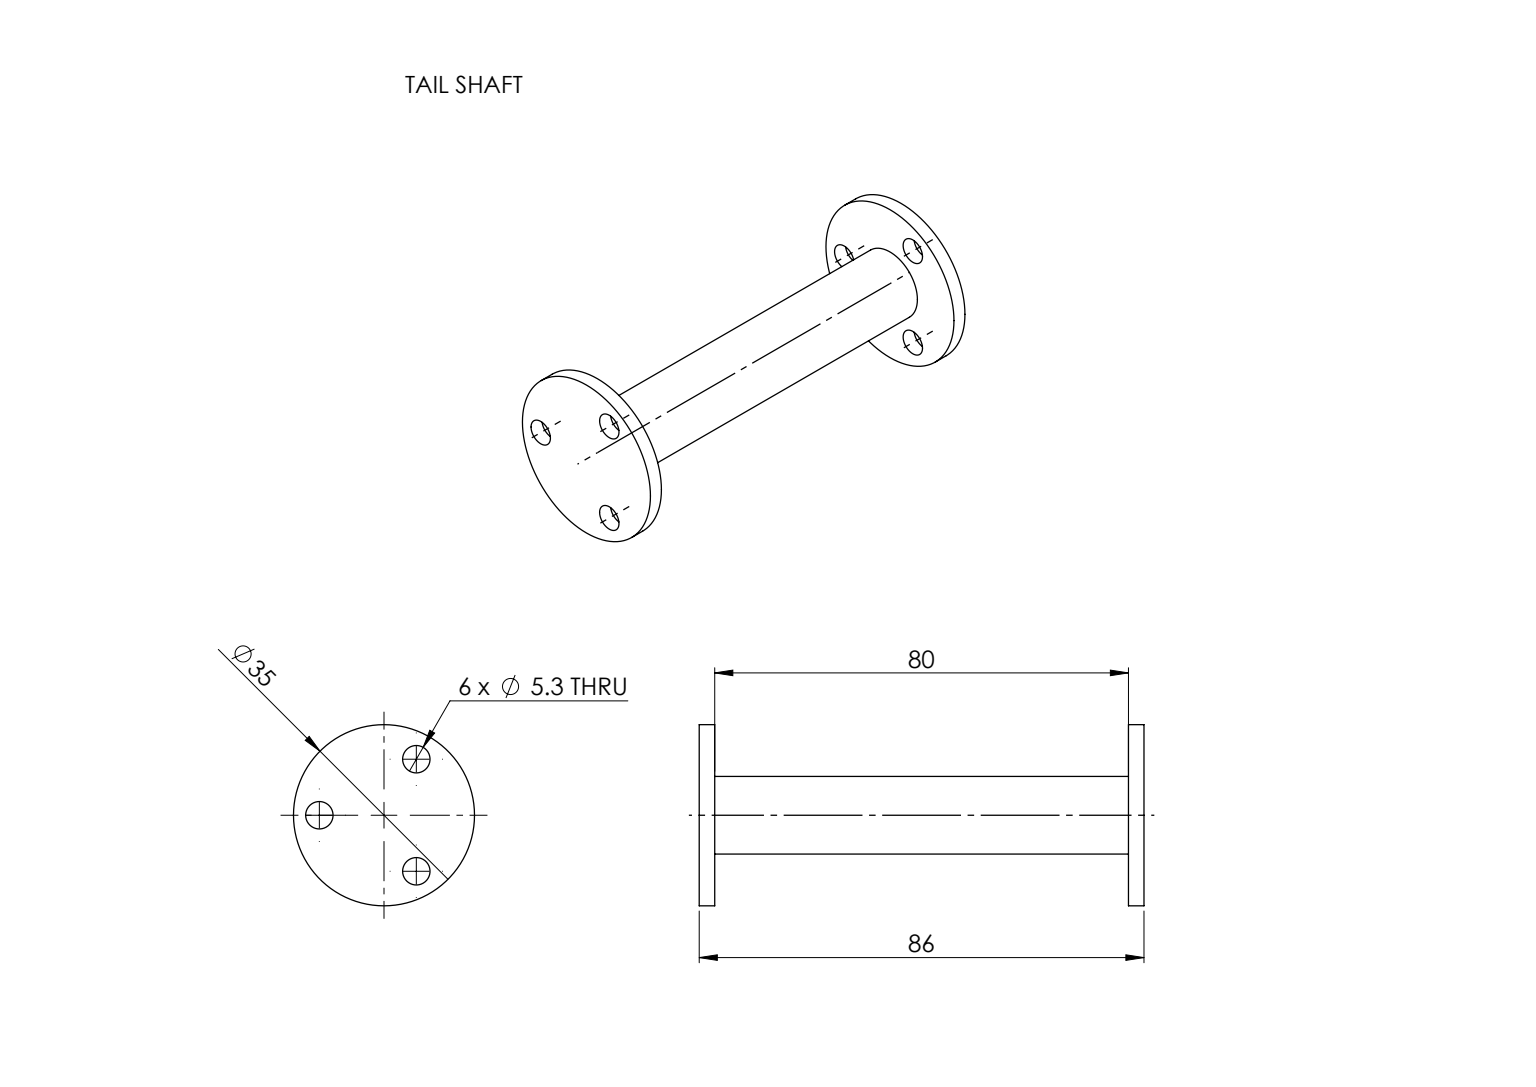
ISO-10303-21;
HEADER;
FILE_DESCRIPTION (('STEP AP214'),
    '1' );
FILE_NAME ('tail shaft.step',
    '2026-10-03T12:29:21',
    ( '' ),
    ( '' ),
    'SwSTEP 2.0',
    'SolidWorks 2026',
    '' );
FILE_SCHEMA (( 'AUTOMOTIVE_DESIGN' ));
ENDSEC;

DATA;
#68=( GEOMETRIC_REPRESENTATION_CONTEXT ( 3 ) GLOBAL_UNCERTAINTY_ASSIGNED_CONTEXT ( ( #15146 ) ) GLOBAL_UNIT_ASSIGNED_CONTEXT ( ( #18068, #7816, #19263 ) ) REPRESENTATION_CONTEXT ( 'NONE', 'WORKASPACE' ) );
#77=CARTESIAN_POINT ( 'NONE',  ( -7.500000000000000000, 0.000000000000000000, 126.0000000000000000 ) ) ;
#92=ORIENTED_EDGE ( 'NONE', *, *, #14677, .F. ) ;
#111=PLANE ( 'NONE',  #12445 ) ;
#139=ORIENTED_EDGE ( 'NONE', *, *, #678, .F. ) ;
#155=DIRECTION ( 'NONE',  ( -1.000000000000000000, 0.000000000000000000, 0.000000000000000000 ) ) ;
#169=LINE ( 'NONE', #3246, #19204 ) ;
#185=DIRECTION ( 'NONE',  ( 1.000000000000000000, 0.000000000000000000, 0.000000000000000000 ) ) ;
#190=CIRCLE ( 'NONE', #11381, 7.500000000000000000 ) ;
#191=ORIENTED_EDGE ( 'NONE', *, *, #7409, .T. ) ;
#219=CYLINDRICAL_SURFACE ( 'NONE', #12266, 2.649999999999992806 ) ;
#233=DIRECTION ( 'NONE',  ( 1.000000000000000000, 0.000000000000000000, 0.000000000000000000 ) ) ;
#258=CIRCLE ( 'NONE', #12801, 17.50000000000000355 ) ;
#306=VERTEX_POINT ( 'NONE', #7710 ) ;
#427=DIRECTION ( 'NONE',  ( -0.000000000000000000, -0.000000000000000000, 1.000000000000000000 ) ) ;
#452=DIRECTION ( 'NONE',  ( 1.000000000000000000, 0.000000000000000000, 0.000000000000000000 ) ) ;
#466=CARTESIAN_POINT ( 'NONE',  ( 6.250000000000054179, 10.82531754730546147, 126.0000000000000000 ) ) ;
#469=ORIENTED_EDGE ( 'NONE', *, *, #6864, .F. ) ;
#500=PRODUCT_CONTEXT ( 'NONE', #4657, 'mechanical' ) ;
#505=CARTESIAN_POINT ( 'NONE',  ( 6.249999999999902300, -10.82531754730554496, 126.0000000000000000 ) ) ;
#521=DIRECTION ( 'NONE',  ( -0.000000000000000000, -0.000000000000000000, 1.000000000000000000 ) ) ;
#536=CARTESIAN_POINT ( 'NONE',  ( 0.000000000000000000, 0.000000000000000000, 126.0000000000000000 ) ) ;
#624=EDGE_CURVE ( 'NONE', #15909, #5939, #1544, .T. ) ;
#627=DIRECTION ( 'NONE',  ( -0.000000000000000000, -0.000000000000000000, -1.000000000000000000 ) ) ;
#674=CARTESIAN_POINT ( 'NONE',  ( -15.14999999999999325, 0.000000000000000000, 126.0000000000000000 ) ) ;
#678=EDGE_CURVE ( 'NONE', #18976, #13722, #3439, .T. ) ;
#703=DIRECTION ( 'NONE',  ( 1.000000000000000000, 0.000000000000000000, 0.000000000000000000 ) ) ;
#725=PRODUCT_DEFINITION_CONTEXT ( 'detailed design', #8064, 'design' ) ;
#804=ORIENTED_EDGE ( 'NONE', *, *, #7119, .F. ) ;
#890=CARTESIAN_POINT ( 'NONE',  ( 0.000000000000000000, 0.000000000000000000, 46.00000000000000711 ) ) ;
#892=CIRCLE ( 'NONE', #10354, 2.649999999999987477 ) ;
#937=PLANE ( 'NONE',  #1249 ) ;
#947=ORIENTED_EDGE ( 'NONE', *, *, #16251, .T. ) ;
#971=DIRECTION ( 'NONE',  ( 1.000000000000000000, 0.000000000000000000, 0.000000000000000000 ) ) ;
#975=CARTESIAN_POINT ( 'NONE',  ( -17.50000000000000355, 0.000000000000000000, 43.00000000000000000 ) ) ;
#983=DIRECTION ( 'NONE',  ( 1.000000000000000000, 0.000000000000000000, 0.000000000000000000 ) ) ;
#1033=ORIENTED_EDGE ( 'NONE', *, *, #9203, .T. ) ;
#1066=ADVANCED_FACE ( 'NONE', ( #20892 ), #9764, .F. ) ;
#1081=DIRECTION ( 'NONE',  ( 1.000000000000000000, 0.000000000000000000, 0.000000000000000000 ) ) ;
#1082=AXIS2_PLACEMENT_3D ( 'NONE', #19195, #7847, #1081 ) ;
#1101=DIRECTION ( 'NONE',  ( 0.000000000000000000, 0.000000000000000000, 1.000000000000000000 ) ) ;
#1103=EDGE_CURVE ( 'NONE', #4018, #1536, #6170, .T. ) ;
#1116=VERTEX_POINT ( 'NONE', #13564 ) ;
#1131=CIRCLE ( 'NONE', #2124, 7.500000000000000000 ) ;
#1132=ORIENTED_EDGE ( 'NONE', *, *, #20108, .T. ) ;
#1134=EDGE_CURVE ( 'NONE', #14374, #16949, #2327, .T. ) ;
#1236=ORIENTED_EDGE ( 'NONE', *, *, #16218, .F. ) ;
#1249=AXIS2_PLACEMENT_3D ( 'NONE', #17251, #13857, #4209 ) ;
#1262=LINE ( 'NONE', #15866, #6665 ) ;
#1285=ADVANCED_FACE ( 'NONE', ( #16853 ), #219, .F. ) ;
#1288=DIRECTION ( 'NONE',  ( 0.000000000000000000, 0.000000000000000000, -1.000000000000000000 ) ) ;
#1427=DIRECTION ( 'NONE',  ( -0.000000000000000000, -0.000000000000000000, -1.000000000000000000 ) ) ;
#1474=CARTESIAN_POINT ( 'NONE',  ( -9.850000000000012079, 3.245314017740477087E-16, 129.0000000000000000 ) ) ;
#1514=CARTESIAN_POINT ( 'NONE',  ( 8.899999999999895550, -10.82531754730554496, 126.0000000000000000 ) ) ;
#1520=ORIENTED_EDGE ( 'NONE', *, *, #10012, .F. ) ;
#1526=LINE ( 'NONE', #20792, #14248 ) ;
#1536=VERTEX_POINT ( 'NONE', #9739 ) ;
#1544=LINE ( 'NONE', #17949, #7850 ) ;
#1579=FILL_AREA_STYLE ('',( #14294 ) ) ;
#1593=ORIENTED_EDGE ( 'NONE', *, *, #12629, .T. ) ;
#1629=EDGE_CURVE ( 'NONE', #9402, #16949, #2802, .T. ) ;
#1709=FACE_BOUND ( 'NONE', #7019, .T. ) ;
#1729=CARTESIAN_POINT ( 'NONE',  ( 6.250000000000054179, 10.82531754730546147, 129.0000000000000000 ) ) ;
#1812=DIRECTION ( 'NONE',  ( 1.000000000000000000, 0.000000000000000000, 0.000000000000000000 ) ) ;
#1852=DIRECTION ( 'NONE',  ( 1.000000000000000000, 0.000000000000000000, 0.000000000000000000 ) ) ;
#1863=ADVANCED_BREP_SHAPE_REPRESENTATION ( '', ( #17573, #12461 ), #3268 ) ;
#1912=EDGE_LOOP ( 'NONE', ( #92, #14154 ) ) ;
#1945=ORIENTED_EDGE ( 'NONE', *, *, #16251, .F. ) ;
#1957=PRESENTATION_STYLE_ASSIGNMENT (( #7928 ) ) ;
#1965=EDGE_LOOP ( 'NONE', ( #16112, #3916 ) ) ;
#1966=DIRECTION ( 'NONE',  ( -0.000000000000000000, -0.000000000000000000, 1.000000000000000000 ) ) ;
#2005=VERTEX_POINT ( 'NONE', #3119 ) ;
#2027=VERTEX_POINT ( 'NONE', #19327 ) ;
#2040=FACE_OUTER_BOUND ( 'NONE', #14555, .T. ) ;
#2061=DIRECTION ( 'NONE',  ( 1.000000000000000000, 0.000000000000000000, 0.000000000000000000 ) ) ;
#2124=AXIS2_PLACEMENT_3D ( 'NONE', #16818, #3872, #703 ) ;
#2156=CARTESIAN_POINT ( 'NONE',  ( 0.000000000000000000, 0.000000000000000000, 46.00000000000000711 ) ) ;
#2166=DIRECTION ( 'NONE',  ( 1.000000000000000000, 0.000000000000000000, 0.000000000000000000 ) ) ;
#2253=CARTESIAN_POINT ( 'NONE',  ( 0.000000000000000000, 0.000000000000000000, 126.0000000000000000 ) ) ;
#2257=EDGE_LOOP ( 'NONE', ( #11256, #17039 ) ) ;
#2259=ORIENTED_EDGE ( 'NONE', *, *, #8793, .T. ) ;
#2301=CARTESIAN_POINT ( 'NONE',  ( 6.249999999999902300, -10.82531754730554496, 43.00000000000000000 ) ) ;
#2327=LINE ( 'NONE', #16742, #14309 ) ;
#2341=PRESENTATION_STYLE_ASSIGNMENT (( #17191 ) ) ;
#2375=CYLINDRICAL_SURFACE ( 'NONE', #9838, 2.649999999999993694 ) ;
#2391=DIRECTION ( 'NONE',  ( 1.000000000000000000, 0.000000000000000000, 0.000000000000000000 ) ) ;
#2411=EDGE_LOOP ( 'NONE', ( #5675, #4612, #5419, #5529 ) ) ;
#2456=VERTEX_POINT ( 'NONE', #16330 ) ;
#2461=AXIS2_PLACEMENT_3D ( 'NONE', #20283, #17008, #3365 ) ;
#2485=CARTESIAN_POINT ( 'NONE',  ( 8.899999999999890221, -10.82531754730554496, 46.00000000000000711 ) ) ;
#2527=EDGE_LOOP ( 'NONE', ( #15680, #10668 ) ) ;
#2532=DIRECTION ( 'NONE',  ( 1.000000000000000000, 0.000000000000000000, 0.000000000000000000 ) ) ;
#2559=SURFACE_SIDE_STYLE ('',( #4246 ) ) ;
#2584=LINE ( 'NONE', #10646, #10427 ) ;
#2592=AXIS2_PLACEMENT_3D ( 'NONE', #20669, #17198, #983 ) ;
#2639=CIRCLE ( 'NONE', #8049, 2.649999999999987477 ) ;
#2727=ORIENTED_EDGE ( 'NONE', *, *, #20108, .F. ) ;
#2733=LINE ( 'NONE', #15662, #16649 ) ;
#2793=CARTESIAN_POINT ( 'NONE',  ( 17.50000000000000355, 2.143131898507868643E-15, 46.00000000000000711 ) ) ;
#2802=CIRCLE ( 'NONE', #2461, 2.649999999999987477 ) ;
#2831=FACE_BOUND ( 'NONE', #9265, .T. ) ;
#2836=AXIS2_PLACEMENT_3D ( 'NONE', #11379, #9882, #17856 ) ;
#2886=ORIENTED_EDGE ( 'NONE', *, *, #6253, .T. ) ;
#2893=ORIENTED_EDGE ( 'NONE', *, *, #5507, .F. ) ;
#2899=CARTESIAN_POINT ( 'NONE',  ( 6.250000000000054179, 10.82531754730546147, 43.00000000000000000 ) ) ;
#2922=CARTESIAN_POINT ( 'NONE',  ( 0.000000000000000000, 0.000000000000000000, 46.00000000000000711 ) ) ;
#2941=DIRECTION ( 'NONE',  ( 1.000000000000000000, 0.000000000000000000, 0.000000000000000000 ) ) ;
#2974=CARTESIAN_POINT ( 'NONE',  ( 6.249999999999902300, -10.82531754730554496, 129.0000000000000000 ) ) ;
#2997=EDGE_LOOP ( 'NONE', ( #1593, #20208 ) ) ;
#3000=CARTESIAN_POINT ( 'NONE',  ( -7.500000000000000000, 0.000000000000000000, 126.0000000000000000 ) ) ;
#3007=LINE ( 'NONE', #2793, #5192 ) ;
#3008=VERTEX_POINT ( 'NONE', #19183 ) ;
#3074=AXIS2_PLACEMENT_3D ( 'NONE', #466, #9793, #4921 ) ;
#3119=CARTESIAN_POINT ( 'NONE',  ( 3.600000000000066702, 10.82531754730546147, 46.00000000000000711 ) ) ;
#3210=CARTESIAN_POINT ( 'NONE',  ( -12.50000000000000533, 0.000000000000000000, 43.00000000000000000 ) ) ;
#3246=CARTESIAN_POINT ( 'NONE',  ( -17.50000000000000355, 2.143131898507868643E-15, 126.0000000000000000 ) ) ;
#3255=CIRCLE ( 'NONE', #17825, 17.50000000000000355 ) ;
#3261=CIRCLE ( 'NONE', #13748, 17.50000000000000355 ) ;
#3268=( GEOMETRIC_REPRESENTATION_CONTEXT ( 3 ) GLOBAL_UNCERTAINTY_ASSIGNED_CONTEXT ( ( #3689 ) ) GLOBAL_UNIT_ASSIGNED_CONTEXT ( ( #10185, #9871, #10087 ) ) REPRESENTATION_CONTEXT ( 'NONE', 'WORKASPACE' ) );
#3333=CYLINDRICAL_SURFACE ( 'NONE', #3074, 2.649999999999993694 ) ;
#3359=ORIENTED_EDGE ( 'NONE', *, *, #9567, .T. ) ;
#3361=DIRECTION ( 'NONE',  ( 0.000000000000000000, 0.000000000000000000, 1.000000000000000000 ) ) ;
#3365=DIRECTION ( 'NONE',  ( -1.000000000000000000, 0.000000000000000000, 0.000000000000000000 ) ) ;
#3374=EDGE_CURVE ( 'NONE', #19870, #7692, #14900, .T. ) ;
#3408=DIRECTION ( 'NONE',  ( -1.000000000000000000, 0.000000000000000000, 0.000000000000000000 ) ) ;
#3430=CARTESIAN_POINT ( 'NONE',  ( 6.250000000000054179, 10.82531754730546147, 129.0000000000000000 ) ) ;
#3439=CIRCLE ( 'NONE', #12930, 7.500000000000000000 ) ;
#3440=EDGE_LOOP ( 'NONE', ( #8664, #8272 ) ) ;
#3444=ORIENTED_EDGE ( 'NONE', *, *, #12629, .F. ) ;
#3467=VERTEX_POINT ( 'NONE', #19566 ) ;
#3481=EDGE_CURVE ( 'NONE', #14374, #14158, #20407, .T. ) ;
#3484=VECTOR ( 'NONE', #15619, 1000.000000000000000 ) ;
#3485=FACE_OUTER_BOUND ( 'NONE', #2527, .T. ) ;
#3500=EDGE_LOOP ( 'NONE', ( #2727, #10830, #6356, #14645 ) ) ;
#3548=ORIENTED_EDGE ( 'NONE', *, *, #15150, .T. ) ;
#3549=CARTESIAN_POINT ( 'NONE',  ( 0.000000000000000000, 0.000000000000000000, 43.00000000000000000 ) ) ;
#3621=DIRECTION ( 'NONE',  ( -1.000000000000000000, 0.000000000000000000, 0.000000000000000000 ) ) ;
#3658=ORIENTED_EDGE ( 'NONE', *, *, #1134, .F. ) ;
#3689=UNCERTAINTY_MEASURE_WITH_UNIT (LENGTH_MEASURE( 1.000000000000000082E-05 ), #10185, 'distance_accuracy_value', 'NONE');
#3849=EDGE_LOOP ( 'NONE', ( #17467, #17599, #2886, #15674 ) ) ;
#3872=DIRECTION ( 'NONE',  ( 0.000000000000000000, 0.000000000000000000, 1.000000000000000000 ) ) ;
#3916=ORIENTED_EDGE ( 'NONE', *, *, #3481, .T. ) ;
#3919=ADVANCED_FACE ( 'NONE', ( #17957 ), #3333, .F. ) ;
#3940=AXIS2_PLACEMENT_3D ( 'NONE', #15189, #10205, #12117 ) ;
#3947=DIRECTION ( 'NONE',  ( -1.000000000000000000, 0.000000000000000000, 0.000000000000000000 ) ) ;
#3950=FACE_OUTER_BOUND ( 'NONE', #17672, .T. ) ;
#3992=LINE ( 'NONE', #15233, #8841 ) ;
#4018=VERTEX_POINT ( 'NONE', #5639 ) ;
#4174=CARTESIAN_POINT ( 'NONE',  ( 0.000000000000000000, 0.000000000000000000, 126.0000000000000000 ) ) ;
#4194=EDGE_CURVE ( 'NONE', #3467, #17864, #1526, .T. ) ;
#4209=DIRECTION ( 'NONE',  ( 1.000000000000000000, 0.000000000000000000, -0.000000000000000000 ) ) ;
#4228=CYLINDRICAL_SURFACE ( 'NONE', #20218, 7.500000000000000000 ) ;
#4246=SURFACE_STYLE_FILL_AREA ( #20248 ) ;
#4331=AXIS2_PLACEMENT_3D ( 'NONE', #13440, #5151, #5053 ) ;
#4340=DIRECTION ( 'NONE',  ( -0.000000000000000000, -0.000000000000000000, -1.000000000000000000 ) ) ;
#4386=CYLINDRICAL_SURFACE ( 'NONE', #12999, 2.649999999999994582 ) ;
#4453=EDGE_CURVE ( 'NONE', #4018, #1116, #8381, .T. ) ;
#4486=DIRECTION ( 'NONE',  ( 0.000000000000000000, 0.000000000000000000, 1.000000000000000000 ) ) ;
#4524=ORIENTED_EDGE ( 'NONE', *, *, #7812, .T. ) ;
#4571=CIRCLE ( 'NONE', #11339, 17.50000000000000355 ) ;
#4598=CARTESIAN_POINT ( 'NONE',  ( 8.900000000000041211, 10.82531754730546147, 46.00000000000000711 ) ) ;
#4612=ORIENTED_EDGE ( 'NONE', *, *, #9538, .T. ) ;
#4657=APPLICATION_CONTEXT ( 'automotive_design' ) ;
#4703=DIRECTION ( 'NONE',  ( -1.000000000000000000, 0.000000000000000000, 0.000000000000000000 ) ) ;
#4708=CARTESIAN_POINT ( 'NONE',  ( 3.599999999999909051, -10.82531754730554496, 46.00000000000000711 ) ) ;
#4720=EDGE_CURVE ( 'NONE', #19863, #18058, #20338, .T. ) ;
#4734=EDGE_CURVE ( 'NONE', #8346, #8326, #11537, .T. ) ;
#4768=CARTESIAN_POINT ( 'NONE',  ( 3.600000000000060485, 10.82531754730546147, 46.00000000000000711 ) ) ;
#4777=ORIENTED_EDGE ( 'NONE', *, *, #13561, .T. ) ;
#4782=AXIS2_PLACEMENT_3D ( 'NONE', #2974, #5936, #17283 ) ;
#4829=VECTOR ( 'NONE', #5253, 1000.000000000000000 ) ;
#4921=DIRECTION ( 'NONE',  ( -1.000000000000000000, 0.000000000000000000, 0.000000000000000000 ) ) ;
#4940=EDGE_CURVE ( 'NONE', #16324, #17864, #18668, .T. ) ;
#4956=AXIS2_PLACEMENT_3D ( 'NONE', #10582, #521, #2532 ) ;
#4964=EDGE_CURVE ( 'NONE', #18976, #14272, #3992, .T. ) ;
#5028=DIRECTION ( 'NONE',  ( -0.000000000000000000, -0.000000000000000000, -1.000000000000000000 ) ) ;
#5053=DIRECTION ( 'NONE',  ( 1.000000000000000000, 0.000000000000000000, 0.000000000000000000 ) ) ;
#5151=DIRECTION ( 'NONE',  ( -0.000000000000000000, -0.000000000000000000, 1.000000000000000000 ) ) ;
#5154=VECTOR ( 'NONE', #19469, 1000.000000000000000 ) ;
#5192=VECTOR ( 'NONE', #6070, 1000.000000000000000 ) ;
#5232=CIRCLE ( 'NONE', #9294, 2.649999999999994582 ) ;
#5253=DIRECTION ( 'NONE',  ( -0.000000000000000000, -0.000000000000000000, 1.000000000000000000 ) ) ;
#5258=PRODUCT_DEFINITION_SHAPE ( 'NONE', 'NONE',  #17526 ) ;
#5351=FACE_OUTER_BOUND ( 'NONE', #17125, .T. ) ;
#5395=DIRECTION ( 'NONE',  ( 1.000000000000000000, 0.000000000000000000, 0.000000000000000000 ) ) ;
#5403=ORIENTED_EDGE ( 'NONE', *, *, #4453, .T. ) ;
#5419=ORIENTED_EDGE ( 'NONE', *, *, #10012, .T. ) ;
#5431=DIRECTION ( 'NONE',  ( -0.000000000000000000, -0.000000000000000000, -1.000000000000000000 ) ) ;
#5507=EDGE_CURVE ( 'NONE', #16541, #16592, #12657, .T. ) ;
#5529=ORIENTED_EDGE ( 'NONE', *, *, #624, .F. ) ;
#5535=AXIS2_PLACEMENT_3D ( 'NONE', #2899, #4486, #10848 ) ;
#5627=AXIS2_PLACEMENT_3D ( 'NONE', #16922, #10149, #10466 ) ;
#5639=CARTESIAN_POINT ( 'NONE',  ( 17.50000000000000355, 0.000000000000000000, 126.0000000000000000 ) ) ;
#5644=AXIS2_PLACEMENT_3D ( 'NONE', #19883, #18290, #2391 ) ;
#5675=ORIENTED_EDGE ( 'NONE', *, *, #13509, .F. ) ;
#5708=CARTESIAN_POINT ( 'NONE',  ( -12.50000000000000533, 0.000000000000000000, 46.00000000000000711 ) ) ;
#5720=FILL_AREA_STYLE_COLOUR ( '', #11738 ) ;
#5729=EDGE_CURVE ( 'NONE', #10676, #2005, #892, .T. ) ;
#5753=CYLINDRICAL_SURFACE ( 'NONE', #18979, 17.50000000000000355 ) ;
#5773=CARTESIAN_POINT ( 'NONE',  ( 8.899999999999895550, -10.82531754730554496, 46.00000000000000711 ) ) ;
#5812=AXIS2_PLACEMENT_3D ( 'NONE', #3210, #18222, #6384 ) ;
#5866=DIRECTION ( 'NONE',  ( 0.000000000000000000, 0.000000000000000000, 1.000000000000000000 ) ) ;
#5871=EDGE_CURVE ( 'NONE', #18341, #1116, #3261, .T. ) ;
#5873=ORIENTED_EDGE ( 'NONE', *, *, #10339, .T. ) ;
#5936=DIRECTION ( 'NONE',  ( 0.000000000000000000, 0.000000000000000000, -1.000000000000000000 ) ) ;
#5939=VERTEX_POINT ( 'NONE', #975 ) ;
#5947=DIRECTION ( 'NONE',  ( 1.000000000000000000, 0.000000000000000000, 0.000000000000000000 ) ) ;
#5955=AXIS2_PLACEMENT_3D ( 'NONE', #16796, #7041, #16904 ) ;
#5975=CIRCLE ( 'NONE', #2592, 2.649999999999987477 ) ;
#5980=ORIENTED_EDGE ( 'NONE', *, *, #9203, .F. ) ;
#6013=FACE_OUTER_BOUND ( 'NONE', #6879, .T. ) ;
#6065=VERTEX_POINT ( 'NONE', #14006 ) ;
#6066=DIRECTION ( 'NONE',  ( -0.000000000000000000, -0.000000000000000000, 1.000000000000000000 ) ) ;
#6070=DIRECTION ( 'NONE',  ( -0.000000000000000000, -0.000000000000000000, -1.000000000000000000 ) ) ;
#6073=DIRECTION ( 'NONE',  ( 1.000000000000000000, 0.000000000000000000, 0.000000000000000000 ) ) ;
#6170=CIRCLE ( 'NONE', #15638, 17.50000000000000355 ) ;
#6176=AXIS2_PLACEMENT_3D ( 'NONE', #2301, #19890, #10350 ) ;
#6253=EDGE_CURVE ( 'NONE', #2005, #10676, #18503, .T. ) ;
#6282=DIRECTION ( 'NONE',  ( -1.000000000000000000, 0.000000000000000000, 0.000000000000000000 ) ) ;
#6322=MECHANICAL_DESIGN_GEOMETRIC_PRESENTATION_REPRESENTATION('',(#17505),#17165);
#6344=EDGE_CURVE ( 'NONE', #2456, #306, #10039, .T. ) ;
#6356=ORIENTED_EDGE ( 'NONE', *, *, #4194, .T. ) ;
#6371=DIRECTION ( 'NONE',  ( -0.000000000000000000, -0.000000000000000000, -1.000000000000000000 ) ) ;
#6384=DIRECTION ( 'NONE',  ( 1.000000000000000000, 0.000000000000000000, 0.000000000000000000 ) ) ;
#6433=CARTESIAN_POINT ( 'NONE',  ( 8.899999999999895550, -10.82531754730554496, 43.00000000000000000 ) ) ;
#6487=MECHANICAL_DESIGN_GEOMETRIC_PRESENTATION_REPRESENTATION('',(#12939),#68);
#6510=DIRECTION ( 'NONE',  ( 1.000000000000000000, 0.000000000000000000, 0.000000000000000000 ) ) ;
#6519=CIRCLE ( 'NONE', #6176, 2.649999999999993694 ) ;
#6665=VECTOR ( 'NONE', #12583, 1000.000000000000000 ) ;
#6671=CIRCLE ( 'NONE', #15488, 17.50000000000000355 ) ;
#6678=CARTESIAN_POINT ( 'NONE',  ( 6.250000000000054179, 10.82531754730546147, 46.00000000000000711 ) ) ;
#6689=DIRECTION ( 'NONE',  ( -0.000000000000000000, -0.000000000000000000, 1.000000000000000000 ) ) ;
#6722=EDGE_LOOP ( 'NONE', ( #8234, #10105, #11324, #2893 ) ) ;
#6728=EDGE_LOOP ( 'NONE', ( #18108, #11843, #4524, #13099 ) ) ;
#6731=DIRECTION ( 'NONE',  ( 0.000000000000000000, 0.000000000000000000, -1.000000000000000000 ) ) ;
#6742=AXIS2_PLACEMENT_3D ( 'NONE', #16483, #1966, #2061 ) ;
#6765=EDGE_CURVE ( 'NONE', #1116, #18341, #14794, .T. ) ;
#6771=FACE_BOUND ( 'NONE', #8303, .T. ) ;
#6860=ORIENTED_EDGE ( 'NONE', *, *, #8907, .F. ) ;
#6864=EDGE_CURVE ( 'NONE', #15909, #6065, #258, .T. ) ;
#6869=UNCERTAINTY_MEASURE_WITH_UNIT (LENGTH_MEASURE( 1.000000000000000082E-05 ), #20342, 'distance_accuracy_value', 'NONE');
#6879=EDGE_LOOP ( 'NONE', ( #19920, #12113 ) ) ;
#6929=CARTESIAN_POINT ( 'NONE',  ( 6.249999999999902300, -10.82531754730554496, 126.0000000000000000 ) ) ;
#6942=ORIENTED_EDGE ( 'NONE', *, *, #18612, .T. ) ;
#6951=DIRECTION ( 'NONE',  ( -1.000000000000000000, 0.000000000000000000, 0.000000000000000000 ) ) ;
#7019=EDGE_LOOP ( 'NONE', ( #8213, #17767 ) ) ;
#7030=DIRECTION ( 'NONE',  ( -0.000000000000000000, -0.000000000000000000, -1.000000000000000000 ) ) ;
#7036=CARTESIAN_POINT ( 'NONE',  ( -9.850000000000019185, 0.000000000000000000, 46.00000000000000711 ) ) ;
#7041=DIRECTION ( 'NONE',  ( -0.000000000000000000, -0.000000000000000000, 1.000000000000000000 ) ) ;
#7095=EDGE_CURVE ( 'NONE', #14158, #9402, #8107, .T. ) ;
#7119=EDGE_CURVE ( 'NONE', #17864, #16324, #2639, .T. ) ;
#7120=EDGE_CURVE ( 'NONE', #1536, #4018, #6671, .T. ) ;
#7174=ORIENTED_EDGE ( 'NONE', *, *, #7095, .T. ) ;
#7199=ORIENTED_EDGE ( 'NONE', *, *, #9538, .F. ) ;
#7298=PRODUCT ( 'tail shaft', 'tail shaft', '', ( #500 ) ) ;
#7304=FACE_OUTER_BOUND ( 'NONE', #14599, .T. ) ;
#7360=AXIS2_PLACEMENT_3D ( 'NONE', #3549, #1101, #11820 ) ;
#7409=EDGE_CURVE ( 'NONE', #8346, #2456, #2584, .T. ) ;
#7414=CARTESIAN_POINT ( 'NONE',  ( 6.250000000000054179, 10.82531754730546147, 43.00000000000000000 ) ) ;
#7597=CARTESIAN_POINT ( 'NONE',  ( -7.500000000000000000, 0.000000000000000000, 46.00000000000000711 ) ) ;
#7667=AXIS2_PLACEMENT_3D ( 'NONE', #18315, #627, #11752 ) ;
#7692=VERTEX_POINT ( 'NONE', #15350 ) ;
#7710=CARTESIAN_POINT ( 'NONE',  ( 8.899999999999890221, -10.82531754730554496, 126.0000000000000000 ) ) ;
#7795=ORIENTED_EDGE ( 'NONE', *, *, #16233, .T. ) ;
#7812=EDGE_CURVE ( 'NONE', #19863, #10676, #2733, .T. ) ;
#7816=( NAMED_UNIT ( * ) PLANE_ANGLE_UNIT ( ) SI_UNIT ( $, .RADIAN. ) );
#7847=DIRECTION ( 'NONE',  ( 0.000000000000000000, 0.000000000000000000, 1.000000000000000000 ) ) ;
#7850=VECTOR ( 'NONE', #12783, 1000.000000000000000 ) ;
#7928=SURFACE_STYLE_USAGE ( .BOTH. , #16471 ) ;
#7999=EDGE_LOOP ( 'NONE', ( #16814, #1033 ) ) ;
#8049=AXIS2_PLACEMENT_3D ( 'NONE', #19547, #5028, #16363 ) ;
#8064=APPLICATION_CONTEXT ( 'automotive_design' ) ;
#8104=ORIENTED_EDGE ( 'NONE', *, *, #4453, .F. ) ;
#8107=LINE ( 'NONE', #13090, #11437 ) ;
#8160=SHAPE_REPRESENTATION ( 'tail shaft', ( #12461 ), #3268 ) ;
#8172=ORIENTED_EDGE ( 'NONE', *, *, #3481, .F. ) ;
#8181=EDGE_CURVE ( 'NONE', #19870, #16541, #14964, .T. ) ;
#8206=VECTOR ( 'NONE', #15429, 1000.000000000000000 ) ;
#8213=ORIENTED_EDGE ( 'NONE', *, *, #6344, .F. ) ;
#8234=ORIENTED_EDGE ( 'NONE', *, *, #8181, .F. ) ;
#8272=ORIENTED_EDGE ( 'NONE', *, *, #678, .T. ) ;
#8291=CARTESIAN_POINT ( 'NONE',  ( 6.249999999999902300, -10.82531754730554496, 46.00000000000000711 ) ) ;
#8296=CYLINDRICAL_SURFACE ( 'NONE', #11067, 2.649999999999994582 ) ;
#8303=EDGE_LOOP ( 'NONE', ( #804, #9597 ) ) ;
#8326=VERTEX_POINT ( 'NONE', #20110 ) ;
#8346=VERTEX_POINT ( 'NONE', #12070 ) ;
#8380=EDGE_LOOP ( 'NONE', ( #16202, #3359 ) ) ;
#8381=LINE ( 'NONE', #12859, #12916 ) ;
#8511=EDGE_LOOP ( 'NONE', ( #13392, #11486, #2259, #12064 ) ) ;
#8522=EDGE_LOOP ( 'NONE', ( #9035, #9511, #9070, #15038 ) ) ;
#8557=ORIENTED_EDGE ( 'NONE', *, *, #20239, .F. ) ;
#8619=CYLINDRICAL_SURFACE ( 'NONE', #18409, 7.500000000000000000 ) ;
#8633=ORIENTED_EDGE ( 'NONE', *, *, #7409, .F. ) ;
#8646=CYLINDRICAL_SURFACE ( 'NONE', #10245, 2.649999999999993694 ) ;
#8664=ORIENTED_EDGE ( 'NONE', *, *, #11013, .T. ) ;
#8698=CARTESIAN_POINT ( 'NONE',  ( 0.000000000000000000, 0.000000000000000000, 129.0000000000000000 ) ) ;
#8730=DIRECTION ( 'NONE',  ( 1.000000000000000000, 0.000000000000000000, 0.000000000000000000 ) ) ;
#8767=EDGE_LOOP ( 'NONE', ( #19248, #4777 ) ) ;
#8793=EDGE_CURVE ( 'NONE', #13722, #11488, #16390, .T. ) ;
#8826=CARTESIAN_POINT ( 'NONE',  ( 6.249999999999902300, -10.82531754730554496, 126.0000000000000000 ) ) ;
#8841=VECTOR ( 'NONE', #10472, 1000.000000000000000 ) ;
#8872=EDGE_LOOP ( 'NONE', ( #16926, #10022 ) ) ;
#8907=EDGE_CURVE ( 'NONE', #20839, #16808, #18721, .T. ) ;
#8930=DIRECTION ( 'NONE',  ( 1.000000000000000000, 0.000000000000000000, 0.000000000000000000 ) ) ;
#8938=FACE_OUTER_BOUND ( 'NONE', #2411, .T. ) ;
#8947=AXIS2_PLACEMENT_3D ( 'NONE', #890, #7030, #3947 ) ;
#9035=ORIENTED_EDGE ( 'NONE', *, *, #14468, .F. ) ;
#9056=DIRECTION ( 'NONE',  ( -0.000000000000000000, -0.000000000000000000, 1.000000000000000000 ) ) ;
#9070=ORIENTED_EDGE ( 'NONE', *, *, #8907, .T. ) ;
#9115=DIRECTION ( 'NONE',  ( 1.000000000000000000, 0.000000000000000000, 0.000000000000000000 ) ) ;
#9203=EDGE_CURVE ( 'NONE', #2027, #3467, #17727, .T. ) ;
#9265=EDGE_LOOP ( 'NONE', ( #13342, #1945 ) ) ;
#9281=EDGE_LOOP ( 'NONE', ( #13992, #10630, #10058, #8104 ) ) ;
#9291=AXIS2_PLACEMENT_3D ( 'NONE', #8291, #19532, #19625 ) ;
#9294=AXIS2_PLACEMENT_3D ( 'NONE', #18334, #19917, #5395 ) ;
#9298=DIRECTION ( 'NONE',  ( 0.000000000000000000, 0.000000000000000000, 1.000000000000000000 ) ) ;
#9306=FACE_OUTER_BOUND ( 'NONE', #15945, .T. ) ;
#9328=CARTESIAN_POINT ( 'NONE',  ( -15.15000000000000036, 0.000000000000000000, 129.0000000000000000 ) ) ;
#9340=EDGE_CURVE ( 'NONE', #15390, #16808, #9916, .T. ) ;
#9402=VERTEX_POINT ( 'NONE', #674 ) ;
#9467=EDGE_CURVE ( 'NONE', #9747, #20839, #17051, .T. ) ;
#9480=ADVANCED_FACE ( 'NONE', ( #3950 ), #8619, .T. ) ;
#9487=CARTESIAN_POINT ( 'NONE',  ( 0.000000000000000000, 0.000000000000000000, 126.0000000000000000 ) ) ;
#9511=ORIENTED_EDGE ( 'NONE', *, *, #16233, .F. ) ;
#9524=FACE_BOUND ( 'NONE', #7999, .T. ) ;
#9538=EDGE_CURVE ( 'NONE', #6065, #3008, #3007, .T. ) ;
#9567=EDGE_CURVE ( 'NONE', #18058, #19863, #20076, .T. ) ;
#9597=ORIENTED_EDGE ( 'NONE', *, *, #4940, .F. ) ;
#9631=EDGE_CURVE ( 'NONE', #3467, #2027, #12314, .T. ) ;
#9704=ORIENTED_EDGE ( 'NONE', *, *, #7120, .T. ) ;
#9739=CARTESIAN_POINT ( 'NONE',  ( -17.50000000000000355, 2.143131898507868643E-15, 126.0000000000000000 ) ) ;
#9747=VERTEX_POINT ( 'NONE', #18144 ) ;
#9764=CYLINDRICAL_SURFACE ( 'NONE', #12943, 2.649999999999993694 ) ;
#9772=DIRECTION ( 'NONE',  ( -0.000000000000000000, -0.000000000000000000, 1.000000000000000000 ) ) ;
#9793=DIRECTION ( 'NONE',  ( -0.000000000000000000, -0.000000000000000000, -1.000000000000000000 ) ) ;
#9802=CARTESIAN_POINT ( 'NONE',  ( -9.850000000000012079, 0.000000000000000000, 43.00000000000000000 ) ) ;
#9838=AXIS2_PLACEMENT_3D ( 'NONE', #6929, #11810, #18273 ) ;
#9871=( NAMED_UNIT ( * ) PLANE_ANGLE_UNIT ( ) SI_UNIT ( $, .RADIAN. ) );
#9882=DIRECTION ( 'NONE',  ( -0.000000000000000000, -0.000000000000000000, 1.000000000000000000 ) ) ;
#9916=CIRCLE ( 'NONE', #11288, 2.649999999999988365 ) ;
#9957=DIRECTION ( 'NONE',  ( 0.000000000000000000, 0.000000000000000000, -1.000000000000000000 ) ) ;
#9983=DIRECTION ( 'NONE',  ( -0.000000000000000000, -0.000000000000000000, 1.000000000000000000 ) ) ;
#10012=EDGE_CURVE ( 'NONE', #3008, #5939, #16630, .T. ) ;
#10022=ORIENTED_EDGE ( 'NONE', *, *, #19330, .F. ) ;
#10039=CIRCLE ( 'NONE', #7667, 2.649999999999988365 ) ;
#10058=ORIENTED_EDGE ( 'NONE', *, *, #6765, .F. ) ;
#10087=( NAMED_UNIT ( * ) SI_UNIT ( $, .STERADIAN. ) SOLID_ANGLE_UNIT ( ) );
#10090=DIRECTION ( 'NONE',  ( 0.000000000000000000, 0.000000000000000000, -1.000000000000000000 ) ) ;
#10105=ORIENTED_EDGE ( 'NONE', *, *, #3374, .T. ) ;
#10149=DIRECTION ( 'NONE',  ( -0.000000000000000000, -0.000000000000000000, 1.000000000000000000 ) ) ;
#10185=( LENGTH_UNIT ( ) NAMED_UNIT ( * ) SI_UNIT ( .MILLI., .METRE. ) );
#10205=DIRECTION ( 'NONE',  ( 0.000000000000000000, 0.000000000000000000, -1.000000000000000000 ) ) ;
#10214=COLOUR_RGB ( '', 0.40784314, 0.44705882, 0.49803922) ;
#10245=AXIS2_PLACEMENT_3D ( 'NONE', #505, #20197, #6951 ) ;
#10298=CARTESIAN_POINT ( 'NONE',  ( 3.599999999999913936, -10.82531754730554496, 46.00000000000000711 ) ) ;
#10339=EDGE_CURVE ( 'NONE', #5939, #3008, #4571, .T. ) ;
#10350=DIRECTION ( 'NONE',  ( 1.000000000000000000, 0.000000000000000000, 0.000000000000000000 ) ) ;
#10354=AXIS2_PLACEMENT_3D ( 'NONE', #17939, #6689, #233 ) ;
#10394=AXIS2_PLACEMENT_3D ( 'NONE', #13965, #9298, #2941 ) ;
#10427=VECTOR ( 'NONE', #12221, 1000.000000000000000 ) ;
#10448=EDGE_LOOP ( 'NONE', ( #20141, #11591, #14445, #6860 ) ) ;
#10465=ORIENTED_EDGE ( 'NONE', *, *, #6344, .T. ) ;
#10466=DIRECTION ( 'NONE',  ( 1.000000000000000000, 0.000000000000000000, 0.000000000000000000 ) ) ;
#10472=DIRECTION ( 'NONE',  ( -0.000000000000000000, -0.000000000000000000, -1.000000000000000000 ) ) ;
#10524=FACE_BOUND ( 'NONE', #14845, .T. ) ;
#10582=CARTESIAN_POINT ( 'NONE',  ( 6.250000000000054179, 10.82531754730546147, 46.00000000000000711 ) ) ;
#10587=CIRCLE ( 'NONE', #11592, 2.649999999999994582 ) ;
#10600=EDGE_CURVE ( 'NONE', #306, #2456, #14736, .T. ) ;
#10626=CARTESIAN_POINT ( 'NONE',  ( 0.000000000000000000, 0.000000000000000000, 126.0000000000000000 ) ) ;
#10630=ORIENTED_EDGE ( 'NONE', *, *, #20239, .T. ) ;
#10639=PLANE ( 'NONE',  #7360 ) ;
#10646=CARTESIAN_POINT ( 'NONE',  ( 3.599999999999909051, -10.82531754730554496, 126.0000000000000000 ) ) ;
#10668=ORIENTED_EDGE ( 'NONE', *, *, #7120, .F. ) ;
#10676=VERTEX_POINT ( 'NONE', #4598 ) ;
#10705=DIRECTION ( 'NONE',  ( -1.000000000000000000, 0.000000000000000000, 0.000000000000000000 ) ) ;
#10716=ORIENTED_EDGE ( 'NONE', *, *, #10339, .F. ) ;
#10830=ORIENTED_EDGE ( 'NONE', *, *, #9631, .F. ) ;
#10843=CARTESIAN_POINT ( 'NONE',  ( -9.850000000000012079, 0.000000000000000000, 46.00000000000000711 ) ) ;
#10848=DIRECTION ( 'NONE',  ( 1.000000000000000000, 0.000000000000000000, 0.000000000000000000 ) ) ;
#10853=ORIENTED_EDGE ( 'NONE', *, *, #1134, .T. ) ;
#10854=CARTESIAN_POINT ( 'NONE',  ( -12.50000000000000533, 0.000000000000000000, 126.0000000000000000 ) ) ;
#10960=ORIENTED_EDGE ( 'NONE', *, *, #1629, .T. ) ;
#11013=EDGE_CURVE ( 'NONE', #13722, #18976, #190, .T. ) ;
#11067=AXIS2_PLACEMENT_3D ( 'NONE', #11581, #11384, #16557 ) ;
#11095=CARTESIAN_POINT ( 'NONE',  ( 8.900000000000041211, 10.82531754730546147, 126.0000000000000000 ) ) ;
#11242=CARTESIAN_POINT ( 'NONE',  ( 0.000000000000000000, 0.000000000000000000, 126.0000000000000000 ) ) ;
#11256=ORIENTED_EDGE ( 'NONE', *, *, #1629, .F. ) ;
#11288=AXIS2_PLACEMENT_3D ( 'NONE', #20054, #9056, #8730 ) ;
#11324=ORIENTED_EDGE ( 'NONE', *, *, #19330, .T. ) ;
#11339=AXIS2_PLACEMENT_3D ( 'NONE', #17457, #20716, #6510 ) ;
#11353=LINE ( 'NONE', #1514, #16625 ) ;
#11379=CARTESIAN_POINT ( 'NONE',  ( 6.249999999999902300, -10.82531754730554496, 46.00000000000000711 ) ) ;
#11381=AXIS2_PLACEMENT_3D ( 'NONE', #10626, #15806, #5947 ) ;
#11384=DIRECTION ( 'NONE',  ( -0.000000000000000000, -0.000000000000000000, -1.000000000000000000 ) ) ;
#11437=VECTOR ( 'NONE', #19242, 1000.000000000000000 ) ;
#11476=FACE_OUTER_BOUND ( 'NONE', #8522, .T. ) ;
#11486=ORIENTED_EDGE ( 'NONE', *, *, #11013, .F. ) ;
#11488=VERTEX_POINT ( 'NONE', #7597 ) ;
#11537=CIRCLE ( 'NONE', #4782, 2.649999999999993694 ) ;
#11550=DIRECTION ( 'NONE',  ( 1.000000000000000000, 0.000000000000000000, 0.000000000000000000 ) ) ;
#11581=CARTESIAN_POINT ( 'NONE',  ( -12.50000000000000533, 0.000000000000000000, 126.0000000000000000 ) ) ;
#11591=ORIENTED_EDGE ( 'NONE', *, *, #14468, .T. ) ;
#11592=AXIS2_PLACEMENT_3D ( 'NONE', #13438, #12044, #11931 ) ;
#11738=COLOUR_RGB ( '', 0.40784314, 0.44705882, 0.49803922) ;
#11742=CYLINDRICAL_SURFACE ( 'NONE', #5627, 2.649999999999992806 ) ;
#11752=DIRECTION ( 'NONE',  ( -1.000000000000000000, 0.000000000000000000, 0.000000000000000000 ) ) ;
#11810=DIRECTION ( 'NONE',  ( -0.000000000000000000, -0.000000000000000000, -1.000000000000000000 ) ) ;
#11820=DIRECTION ( 'NONE',  ( 1.000000000000000000, 0.000000000000000000, -0.000000000000000000 ) ) ;
#11843=ORIENTED_EDGE ( 'NONE', *, *, #4720, .F. ) ;
#11900=DIRECTION ( 'NONE',  ( -1.000000000000000000, 0.000000000000000000, 0.000000000000000000 ) ) ;
#11931=DIRECTION ( 'NONE',  ( -1.000000000000000000, 0.000000000000000000, 0.000000000000000000 ) ) ;
#11966=FACE_OUTER_BOUND ( 'NONE', #8511, .T. ) ;
#12034=VECTOR ( 'NONE', #6066, 1000.000000000000000 ) ;
#12044=DIRECTION ( 'NONE',  ( 0.000000000000000000, 0.000000000000000000, -1.000000000000000000 ) ) ;
#12064=ORIENTED_EDGE ( 'NONE', *, *, #20183, .T. ) ;
#12070=CARTESIAN_POINT ( 'NONE',  ( 3.599999999999909051, -10.82531754730554496, 129.0000000000000000 ) ) ;
#12071=CARTESIAN_POINT ( 'NONE',  ( -17.50000000000000355, 0.000000000000000000, 46.00000000000000711 ) ) ;
#12113=ORIENTED_EDGE ( 'NONE', *, *, #13509, .T. ) ;
#12117=DIRECTION ( 'NONE',  ( -1.000000000000000000, 0.000000000000000000, 0.000000000000000000 ) ) ;
#12146=ORIENTED_EDGE ( 'NONE', *, *, #6765, .T. ) ;
#12221=DIRECTION ( 'NONE',  ( -0.000000000000000000, -0.000000000000000000, -1.000000000000000000 ) ) ;
#12229=FACE_OUTER_BOUND ( 'NONE', #9281, .T. ) ;
#12246=DIRECTION ( 'NONE',  ( 1.000000000000000000, 0.000000000000000000, 0.000000000000000000 ) ) ;
#12266=AXIS2_PLACEMENT_3D ( 'NONE', #6678, #17276, #18553 ) ;
#12275=DIRECTION ( 'NONE',  ( -0.000000000000000000, -0.000000000000000000, -1.000000000000000000 ) ) ;
#12288=AXIS2_PLACEMENT_3D ( 'NONE', #13319, #6731, #13525 ) ;
#12311=VECTOR ( 'NONE', #19697, 1000.000000000000000 ) ;
#12314=CIRCLE ( 'NONE', #13004, 2.649999999999993694 ) ;
#12377=FACE_BOUND ( 'NONE', #8872, .T. ) ;
#12425=CIRCLE ( 'NONE', #10394, 7.500000000000000000 ) ;
#12445=AXIS2_PLACEMENT_3D ( 'NONE', #11242, #9957, #1812 ) ;
#12454=ORIENTED_EDGE ( 'NONE', *, *, #5729, .F. ) ;
#12461=AXIS2_PLACEMENT_3D ( 'NONE', #19474, #3361, #185 ) ;
#12517=EDGE_LOOP ( 'NONE', ( #13678, #18176, #191, #10465 ) ) ;
#12554=LINE ( 'NONE', #4708, #3484 ) ;
#12583=DIRECTION ( 'NONE',  ( -0.000000000000000000, -0.000000000000000000, -1.000000000000000000 ) ) ;
#12594=DIRECTION ( 'NONE',  ( -1.000000000000000000, 0.000000000000000000, 0.000000000000000000 ) ) ;
#12629=EDGE_CURVE ( 'NONE', #16541, #19870, #5232, .T. ) ;
#12657=LINE ( 'NONE', #10843, #12034 ) ;
#12661=DIRECTION ( 'NONE',  ( -0.000000000000000000, -0.000000000000000000, -1.000000000000000000 ) ) ;
#12728=ADVANCED_FACE ( 'NONE', ( #7304 ), #18444, .F. ) ;
#12783=DIRECTION ( 'NONE',  ( -0.000000000000000000, -0.000000000000000000, -1.000000000000000000 ) ) ;
#12801=AXIS2_PLACEMENT_3D ( 'NONE', #2922, #17129, #12246 ) ;
#12848=FACE_BOUND ( 'NONE', #2257, .T. ) ;
#12859=CARTESIAN_POINT ( 'NONE',  ( 17.50000000000000355, 0.000000000000000000, 126.0000000000000000 ) ) ;
#12861=ORIENTED_EDGE ( 'NONE', *, *, #8793, .F. ) ;
#12864=CARTESIAN_POINT ( 'NONE',  ( -12.50000000000000533, 0.000000000000000000, 126.0000000000000000 ) ) ;
#12916=VECTOR ( 'NONE', #9772, 1000.000000000000000 ) ;
#12930=AXIS2_PLACEMENT_3D ( 'NONE', #2253, #14975, #18155 ) ;
#12939=STYLED_ITEM ( 'NONE', ( #1957 ), #17573 ) ;
#12943=AXIS2_PLACEMENT_3D ( 'NONE', #17614, #6371, #14338 ) ;
#12999=AXIS2_PLACEMENT_3D ( 'NONE', #10854, #15731, #3621 ) ;
#13004=AXIS2_PLACEMENT_3D ( 'NONE', #1729, #10090, #3408 ) ;
#13090=CARTESIAN_POINT ( 'NONE',  ( -15.15000000000000036, 0.000000000000000000, 126.0000000000000000 ) ) ;
#13099=ORIENTED_EDGE ( 'NONE', *, *, #5729, .T. ) ;
#13157=DIRECTION ( 'NONE',  ( -0.000000000000000000, -0.000000000000000000, -1.000000000000000000 ) ) ;
#13195=DIRECTION ( 'NONE',  ( 0.000000000000000000, 0.000000000000000000, -1.000000000000000000 ) ) ;
#13209=CARTESIAN_POINT ( 'NONE',  ( -15.15000000000000036, 3.245314017740478073E-16, 46.00000000000000711 ) ) ;
#13214=ADVANCED_FACE ( 'NONE', ( #12377, #15447, #18738, #2831, #6013 ), #937, .T. ) ;
#13286=ORIENTED_EDGE ( 'NONE', *, *, #10600, .T. ) ;
#13305=FACE_OUTER_BOUND ( 'NONE', #12517, .T. ) ;
#13319=CARTESIAN_POINT ( 'NONE',  ( -12.50000000000000533, 0.000000000000000000, 129.0000000000000000 ) ) ;
#13332=CYLINDRICAL_SURFACE ( 'NONE', #4331, 17.50000000000000355 ) ;
#13342=ORIENTED_EDGE ( 'NONE', *, *, #20183, .F. ) ;
#13392=ORIENTED_EDGE ( 'NONE', *, *, #4964, .F. ) ;
#13423=FACE_BOUND ( 'NONE', #8380, .T. ) ;
#13438=CARTESIAN_POINT ( 'NONE',  ( -12.50000000000000533, 0.000000000000000000, 129.0000000000000000 ) ) ;
#13440=CARTESIAN_POINT ( 'NONE',  ( 0.000000000000000000, 0.000000000000000000, 126.0000000000000000 ) ) ;
#13451=CARTESIAN_POINT ( 'NONE',  ( 6.250000000000054179, 10.82531754730546147, 126.0000000000000000 ) ) ;
#13509=EDGE_CURVE ( 'NONE', #6065, #15909, #3255, .T. ) ;
#13525=DIRECTION ( 'NONE',  ( -1.000000000000000000, 0.000000000000000000, 0.000000000000000000 ) ) ;
#13561=EDGE_CURVE ( 'NONE', #8326, #8346, #17153, .T. ) ;
#13564=CARTESIAN_POINT ( 'NONE',  ( 17.50000000000000355, 0.000000000000000000, 129.0000000000000000 ) ) ;
#13678=ORIENTED_EDGE ( 'NONE', *, *, #17299, .F. ) ;
#13689=SHAPE_REPRESENTATION_RELATIONSHIP ( 'NONE' , 'NONE' ,  #8160, #1863 ) ;
#13722=VERTEX_POINT ( 'NONE', #3000 ) ;
#13748=AXIS2_PLACEMENT_3D ( 'NONE', #8698, #15168, #18453 ) ;
#13796=EDGE_LOOP ( 'NONE', ( #12146, #19956 ) ) ;
#13800=( NAMED_UNIT ( * ) SI_UNIT ( $, .STERADIAN. ) SOLID_ANGLE_UNIT ( ) );
#13857=DIRECTION ( 'NONE',  ( 0.000000000000000000, 0.000000000000000000, 1.000000000000000000 ) ) ;
#13889=ORIENTED_EDGE ( 'NONE', *, *, #9467, .T. ) ;
#13965=CARTESIAN_POINT ( 'NONE',  ( 0.000000000000000000, 0.000000000000000000, 46.00000000000000711 ) ) ;
#13973=EDGE_LOOP ( 'NONE', ( #12454, #14568 ) ) ;
#13992=ORIENTED_EDGE ( 'NONE', *, *, #1103, .T. ) ;
#14006=CARTESIAN_POINT ( 'NONE',  ( 17.50000000000000355, 2.143131898507868643E-15, 46.00000000000000711 ) ) ;
#14035=AXIS2_PLACEMENT_3D ( 'NONE', #12864, #12661, #6282 ) ;
#14154=ORIENTED_EDGE ( 'NONE', *, *, #9340, .F. ) ;
#14158=VERTEX_POINT ( 'NONE', #9328 ) ;
#14248=VECTOR ( 'NONE', #17621, 1000.000000000000000 ) ;
#14251=FACE_OUTER_BOUND ( 'NONE', #15198, .T. ) ;
#14272=VERTEX_POINT ( 'NONE', #20869 ) ;
#14294=FILL_AREA_STYLE_COLOUR ( '', #10214 ) ;
#14309=VECTOR ( 'NONE', #13157, 1000.000000000000000 ) ;
#14313=FACE_BOUND ( 'NONE', #1965, .T. ) ;
#14316=EDGE_LOOP ( 'NONE', ( #8557, #9704, #5403, #20757 ) ) ;
#14338=DIRECTION ( 'NONE',  ( -1.000000000000000000, 0.000000000000000000, 0.000000000000000000 ) ) ;
#14374=VERTEX_POINT ( 'NONE', #1474 ) ;
#14445=ORIENTED_EDGE ( 'NONE', *, *, #9340, .T. ) ;
#14468=EDGE_CURVE ( 'NONE', #9747, #15390, #12554, .T. ) ;
#14555=EDGE_LOOP ( 'NONE', ( #3658, #1236, #7174, #10960 ) ) ;
#14568=ORIENTED_EDGE ( 'NONE', *, *, #6253, .F. ) ;
#14599=EDGE_LOOP ( 'NONE', ( #20938, #3444, #14619, #6942 ) ) ;
#14614=CARTESIAN_POINT ( 'NONE',  ( -15.15000000000000036, 3.245314017740477087E-16, 43.00000000000000000 ) ) ;
#14619=ORIENTED_EDGE ( 'NONE', *, *, #5507, .T. ) ;
#14645=ORIENTED_EDGE ( 'NONE', *, *, #7119, .T. ) ;
#14677=EDGE_CURVE ( 'NONE', #16808, #15390, #20431, .T. ) ;
#14679=AXIS2_PLACEMENT_3D ( 'NONE', #3430, #13195, #155 ) ;
#14691=CARTESIAN_POINT ( 'NONE',  ( 3.600000000000066702, 10.82531754730546147, 126.0000000000000000 ) ) ;
#14736=CIRCLE ( 'NONE', #20827, 2.649999999999988365 ) ;
#14794=CIRCLE ( 'NONE', #5644, 17.50000000000000355 ) ;
#14808=AXIS2_PLACEMENT_3D ( 'NONE', #5708, #18131, #18555 ) ;
#14845=EDGE_LOOP ( 'NONE', ( #7795, #13889 ) ) ;
#14900=LINE ( 'NONE', #13209, #4829 ) ;
#14921=ADVANCED_FACE ( 'NONE', ( #8938 ), #15294, .T. ) ;
#14964=CIRCLE ( 'NONE', #5812, 2.649999999999994582 ) ;
#14969=FACE_OUTER_BOUND ( 'NONE', #10448, .T. ) ;
#14975=DIRECTION ( 'NONE',  ( 0.000000000000000000, 0.000000000000000000, 1.000000000000000000 ) ) ;
#15030=CIRCLE ( 'NONE', #14035, 2.649999999999987477 ) ;
#15038=ORIENTED_EDGE ( 'NONE', *, *, #14677, .T. ) ;
#15146=UNCERTAINTY_MEASURE_WITH_UNIT (LENGTH_MEASURE( 1.000000000000000082E-05 ), #18068, 'distance_accuracy_value', 'NONE');
#15150=EDGE_CURVE ( 'NONE', #16949, #9402, #15030, .T. ) ;
#15168=DIRECTION ( 'NONE',  ( -0.000000000000000000, -0.000000000000000000, 1.000000000000000000 ) ) ;
#15189=CARTESIAN_POINT ( 'NONE',  ( 6.249999999999902300, -10.82531754730554496, 129.0000000000000000 ) ) ;
#15198=EDGE_LOOP ( 'NONE', ( #8172, #10853, #3548, #15377 ) ) ;
#15233=CARTESIAN_POINT ( 'NONE',  ( 7.500000000000000000, 9.184850993605147944E-16, 126.0000000000000000 ) ) ;
#15294=CYLINDRICAL_SURFACE ( 'NONE', #8947, 17.50000000000000355 ) ;
#15338=FACE_OUTER_BOUND ( 'NONE', #6728, .T. ) ;
#15350=CARTESIAN_POINT ( 'NONE',  ( -15.14999999999999325, 3.245314017740474129E-16, 46.00000000000000711 ) ) ;
#15377=ORIENTED_EDGE ( 'NONE', *, *, #7095, .F. ) ;
#15390=VERTEX_POINT ( 'NONE', #10298 ) ;
#15429=DIRECTION ( 'NONE',  ( -0.000000000000000000, -0.000000000000000000, 1.000000000000000000 ) ) ;
#15447=FACE_BOUND ( 'NONE', #13973, .T. ) ;
#15488=AXIS2_PLACEMENT_3D ( 'NONE', #9487, #19443, #1852 ) ;
#15514=DIRECTION ( 'NONE',  ( -0.000000000000000000, -0.000000000000000000, 1.000000000000000000 ) ) ;
#15617=AXIS2_PLACEMENT_3D ( 'NONE', #17047, #12275, #12594 ) ;
#15619=DIRECTION ( 'NONE',  ( -0.000000000000000000, -0.000000000000000000, 1.000000000000000000 ) ) ;
#15638=AXIS2_PLACEMENT_3D ( 'NONE', #536, #427, #11550 ) ;
#15662=CARTESIAN_POINT ( 'NONE',  ( 8.900000000000046541, 10.82531754730546147, 46.00000000000000711 ) ) ;
#15674=ORIENTED_EDGE ( 'NONE', *, *, #7812, .F. ) ;
#15680=ORIENTED_EDGE ( 'NONE', *, *, #1103, .F. ) ;
#15731=DIRECTION ( 'NONE',  ( -0.000000000000000000, -0.000000000000000000, -1.000000000000000000 ) ) ;
#15784=FACE_BOUND ( 'NONE', #8767, .T. ) ;
#15806=DIRECTION ( 'NONE',  ( 0.000000000000000000, 0.000000000000000000, 1.000000000000000000 ) ) ;
#15807=EDGE_CURVE ( 'NONE', #18058, #2005, #16313, .T. ) ;
#15866=CARTESIAN_POINT ( 'NONE',  ( 8.900000000000046541, 10.82531754730546147, 126.0000000000000000 ) ) ;
#15909=VERTEX_POINT ( 'NONE', #12071 ) ;
#15945=EDGE_LOOP ( 'NONE', ( #7199, #469, #18599, #5873 ) ) ;
#16112=ORIENTED_EDGE ( 'NONE', *, *, #16218, .T. ) ;
#16184=EDGE_LOOP ( 'NONE', ( #16538, #20385, #13286, #8633 ) ) ;
#16202=ORIENTED_EDGE ( 'NONE', *, *, #4720, .T. ) ;
#16218=EDGE_CURVE ( 'NONE', #14158, #14374, #10587, .T. ) ;
#16227=ADVANCED_FACE ( 'NONE', ( #18516 ), #8646, .F. ) ;
#16233=EDGE_CURVE ( 'NONE', #20839, #9747, #6519, .T. ) ;
#16251=EDGE_CURVE ( 'NONE', #14272, #11488, #1131, .T. ) ;
#16298=CARTESIAN_POINT ( 'NONE',  ( 8.900000000000046541, 10.82531754730546147, 43.00000000000000000 ) ) ;
#16300=ORIENTED_EDGE ( 'NONE', *, *, #4194, .F. ) ;
#16313=LINE ( 'NONE', #4768, #12311 ) ;
#16324=VERTEX_POINT ( 'NONE', #11095 ) ;
#16330=CARTESIAN_POINT ( 'NONE',  ( 3.599999999999913936, -10.82531754730554496, 126.0000000000000000 ) ) ;
#16363=DIRECTION ( 'NONE',  ( -1.000000000000000000, 0.000000000000000000, 0.000000000000000000 ) ) ;
#16390=LINE ( 'NONE', #77, #5154 ) ;
#16416=PRODUCT_DEFINITION_FORMATION_WITH_SPECIFIED_SOURCE ( 'ANY', '', #7298, .NOT_KNOWN. ) ;
#16450=CYLINDRICAL_SURFACE ( 'NONE', #9291, 2.649999999999993694 ) ;
#16471=SURFACE_SIDE_STYLE ('',( #17583 ) ) ;
#16483=CARTESIAN_POINT ( 'NONE',  ( -12.50000000000000533, 0.000000000000000000, 46.00000000000000711 ) ) ;
#16515=ORIENTED_EDGE ( 'NONE', *, *, #4940, .T. ) ;
#16518=DIRECTION ( 'NONE',  ( -1.000000000000000000, 0.000000000000000000, 0.000000000000000000 ) ) ;
#16520=EDGE_LOOP ( 'NONE', ( #5980, #1132, #16515, #16300 ) ) ;
#16538=ORIENTED_EDGE ( 'NONE', *, *, #13561, .F. ) ;
#16541=VERTEX_POINT ( 'NONE', #9802 ) ;
#16557=DIRECTION ( 'NONE',  ( -1.000000000000000000, 0.000000000000000000, 0.000000000000000000 ) ) ;
#16592=VERTEX_POINT ( 'NONE', #7036 ) ;
#16625=VECTOR ( 'NONE', #17826, 1000.000000000000000 ) ;
#16630=CIRCLE ( 'NONE', #1082, 17.50000000000000355 ) ;
#16649=VECTOR ( 'NONE', #17368, 1000.000000000000000 ) ;
#16664=ADVANCED_FACE ( 'NONE', ( #13305 ), #2375, .F. ) ;
#16735=ADVANCED_FACE ( 'NONE', ( #12229 ), #5753, .T. ) ;
#16742=CARTESIAN_POINT ( 'NONE',  ( -9.850000000000012079, 3.245314017740478073E-16, 126.0000000000000000 ) ) ;
#16796=CARTESIAN_POINT ( 'NONE',  ( -12.50000000000000533, 0.000000000000000000, 46.00000000000000711 ) ) ;
#16808=VERTEX_POINT ( 'NONE', #2485 ) ;
#16814=ORIENTED_EDGE ( 'NONE', *, *, #9631, .T. ) ;
#16818=CARTESIAN_POINT ( 'NONE',  ( 0.000000000000000000, 0.000000000000000000, 46.00000000000000711 ) ) ;
#16853=FACE_OUTER_BOUND ( 'NONE', #3849, .T. ) ;
#16904=DIRECTION ( 'NONE',  ( 1.000000000000000000, 0.000000000000000000, 0.000000000000000000 ) ) ;
#16922=CARTESIAN_POINT ( 'NONE',  ( 6.250000000000054179, 10.82531754730546147, 46.00000000000000711 ) ) ;
#16926=ORIENTED_EDGE ( 'NONE', *, *, #18612, .F. ) ;
#16949=VERTEX_POINT ( 'NONE', #17747 ) ;
#17008=DIRECTION ( 'NONE',  ( -0.000000000000000000, -0.000000000000000000, -1.000000000000000000 ) ) ;
#17039=ORIENTED_EDGE ( 'NONE', *, *, #15150, .F. ) ;
#17047=CARTESIAN_POINT ( 'NONE',  ( 0.000000000000000000, 0.000000000000000000, 46.00000000000000711 ) ) ;
#17051=CIRCLE ( 'NONE', #18756, 2.649999999999993694 ) ;
#17058=ADVANCED_FACE ( 'NONE', ( #14969 ), #19732, .F. ) ;
#17097=FACE_BOUND ( 'NONE', #2997, .T. ) ;
#17125=EDGE_LOOP ( 'NONE', ( #10716, #1520 ) ) ;
#17129=DIRECTION ( 'NONE',  ( 0.000000000000000000, 0.000000000000000000, 1.000000000000000000 ) ) ;
#17153=CIRCLE ( 'NONE', #3940, 2.649999999999993694 ) ;
#17165=( GEOMETRIC_REPRESENTATION_CONTEXT ( 3 ) GLOBAL_UNCERTAINTY_ASSIGNED_CONTEXT ( ( #6869 ) ) GLOBAL_UNIT_ASSIGNED_CONTEXT ( ( #20342, #18887, #13800 ) ) REPRESENTATION_CONTEXT ( 'NONE', 'WORKASPACE' ) );
#17191=SURFACE_STYLE_USAGE ( .BOTH. , #2559 ) ;
#17198=DIRECTION ( 'NONE',  ( -0.000000000000000000, -0.000000000000000000, 1.000000000000000000 ) ) ;
#17251=CARTESIAN_POINT ( 'NONE',  ( 0.000000000000000000, 0.000000000000000000, 46.00000000000000711 ) ) ;
#17276=DIRECTION ( 'NONE',  ( -0.000000000000000000, -0.000000000000000000, 1.000000000000000000 ) ) ;
#17283=DIRECTION ( 'NONE',  ( -1.000000000000000000, 0.000000000000000000, 0.000000000000000000 ) ) ;
#17299=EDGE_CURVE ( 'NONE', #8326, #306, #11353, .T. ) ;
#17368=DIRECTION ( 'NONE',  ( -0.000000000000000000, -0.000000000000000000, 1.000000000000000000 ) ) ;
#17383=CARTESIAN_POINT ( 'NONE',  ( 0.000000000000000000, 0.000000000000000000, 129.0000000000000000 ) ) ;
#17424=ADVANCED_FACE ( 'NONE', ( #9306 ), #18856, .T. ) ;
#17457=CARTESIAN_POINT ( 'NONE',  ( 0.000000000000000000, 0.000000000000000000, 43.00000000000000000 ) ) ;
#17467=ORIENTED_EDGE ( 'NONE', *, *, #9567, .F. ) ;
#17505=STYLED_ITEM ( 'NONE', ( #2341 ), #1863 ) ;
#17526=PRODUCT_DEFINITION ( 'UNKNOWN', '', #16416, #725 ) ;
#17573=MANIFOLD_SOLID_BREP ( 'Mirror1', #18366 ) ;
#17583=SURFACE_STYLE_FILL_AREA ( #1579 ) ;
#17595=FACE_OUTER_BOUND ( 'NONE', #13796, .T. ) ;
#17599=ORIENTED_EDGE ( 'NONE', *, *, #15807, .T. ) ;
#17614=CARTESIAN_POINT ( 'NONE',  ( 6.250000000000054179, 10.82531754730546147, 126.0000000000000000 ) ) ;
#17621=DIRECTION ( 'NONE',  ( -0.000000000000000000, -0.000000000000000000, -1.000000000000000000 ) ) ;
#17672=EDGE_LOOP ( 'NONE', ( #139, #19621, #947, #12861 ) ) ;
#17727=CIRCLE ( 'NONE', #14679, 2.649999999999993694 ) ;
#17747=CARTESIAN_POINT ( 'NONE',  ( -9.850000000000019185, 3.245314017740474129E-16, 126.0000000000000000 ) ) ;
#17767=ORIENTED_EDGE ( 'NONE', *, *, #10600, .F. ) ;
#17825=AXIS2_PLACEMENT_3D ( 'NONE', #2156, #18475, #8930 ) ;
#17826=DIRECTION ( 'NONE',  ( -0.000000000000000000, -0.000000000000000000, -1.000000000000000000 ) ) ;
#17856=DIRECTION ( 'NONE',  ( 1.000000000000000000, 0.000000000000000000, 0.000000000000000000 ) ) ;
#17864=VERTEX_POINT ( 'NONE', #14691 ) ;
#17893=ADVANCED_FACE ( 'NONE', ( #19649 ), #18077, .F. ) ;
#17939=CARTESIAN_POINT ( 'NONE',  ( 6.250000000000054179, 10.82531754730546147, 46.00000000000000711 ) ) ;
#17949=CARTESIAN_POINT ( 'NONE',  ( -17.50000000000000355, 0.000000000000000000, 46.00000000000000711 ) ) ;
#17957=FACE_OUTER_BOUND ( 'NONE', #3500, .T. ) ;
#18058=VERTEX_POINT ( 'NONE', #18812 ) ;
#18068=( LENGTH_UNIT ( ) NAMED_UNIT ( * ) SI_UNIT ( .MILLI., .METRE. ) );
#18077=CYLINDRICAL_SURFACE ( 'NONE', #6742, 2.649999999999994582 ) ;
#18108=ORIENTED_EDGE ( 'NONE', *, *, #15807, .F. ) ;
#18131=DIRECTION ( 'NONE',  ( -0.000000000000000000, -0.000000000000000000, 1.000000000000000000 ) ) ;
#18144=CARTESIAN_POINT ( 'NONE',  ( 3.599999999999909051, -10.82531754730554496, 43.00000000000000000 ) ) ;
#18155=DIRECTION ( 'NONE',  ( 1.000000000000000000, 0.000000000000000000, 0.000000000000000000 ) ) ;
#18166=ADVANCED_FACE ( 'NONE', ( #14251 ), #4386, .F. ) ;
#18176=ORIENTED_EDGE ( 'NONE', *, *, #4734, .F. ) ;
#18178=ADVANCED_FACE ( 'NONE', ( #11476 ), #16450, .F. ) ;
#18222=DIRECTION ( 'NONE',  ( 0.000000000000000000, 0.000000000000000000, 1.000000000000000000 ) ) ;
#18273=DIRECTION ( 'NONE',  ( -1.000000000000000000, 0.000000000000000000, 0.000000000000000000 ) ) ;
#18290=DIRECTION ( 'NONE',  ( -0.000000000000000000, -0.000000000000000000, 1.000000000000000000 ) ) ;
#18311=DIRECTION ( 'NONE',  ( -0.000000000000000000, -0.000000000000000000, -1.000000000000000000 ) ) ;
#18315=CARTESIAN_POINT ( 'NONE',  ( 6.249999999999902300, -10.82531754730554496, 126.0000000000000000 ) ) ;
#18334=CARTESIAN_POINT ( 'NONE',  ( -12.50000000000000533, 0.000000000000000000, 43.00000000000000000 ) ) ;
#18341=VERTEX_POINT ( 'NONE', #18670 ) ;
#18366=CLOSED_SHELL ( 'NONE', ( #18166, #1066, #16227, #16735, #17893, #1285, #17058, #9480, #14921, #17424, #13214, #20382, #20662, #18178, #19947, #12728, #20889, #18778, #19738, #16664, #3919, #19659 ) ) ;
#18409=AXIS2_PLACEMENT_3D ( 'NONE', #19953, #5431, #11900 ) ;
#18444=CYLINDRICAL_SURFACE ( 'NONE', #14808, 2.649999999999994582 ) ;
#18453=DIRECTION ( 'NONE',  ( 1.000000000000000000, 0.000000000000000000, 0.000000000000000000 ) ) ;
#18475=DIRECTION ( 'NONE',  ( 0.000000000000000000, 0.000000000000000000, 1.000000000000000000 ) ) ;
#18503=CIRCLE ( 'NONE', #4956, 2.649999999999987477 ) ;
#18516=FACE_OUTER_BOUND ( 'NONE', #16184, .T. ) ;
#18553=DIRECTION ( 'NONE',  ( 1.000000000000000000, 0.000000000000000000, 0.000000000000000000 ) ) ;
#18555=DIRECTION ( 'NONE',  ( 1.000000000000000000, 0.000000000000000000, 0.000000000000000000 ) ) ;
#18599=ORIENTED_EDGE ( 'NONE', *, *, #624, .T. ) ;
#18612=EDGE_CURVE ( 'NONE', #16592, #7692, #5975, .T. ) ;
#18634=AXIS2_PLACEMENT_3D ( 'NONE', #19623, #9983, #452 ) ;
#18657=AXIS2_PLACEMENT_3D ( 'NONE', #7414, #19084, #971 ) ;
#18668=CIRCLE ( 'NONE', #20691, 2.649999999999987477 ) ;
#18670=CARTESIAN_POINT ( 'NONE',  ( -17.50000000000000355, 2.143131898507868643E-15, 129.0000000000000000 ) ) ;
#18721=LINE ( 'NONE', #5773, #8206 ) ;
#18738=FACE_BOUND ( 'NONE', #1912, .T. ) ;
#18756=AXIS2_PLACEMENT_3D ( 'NONE', #20379, #5866, #2166 ) ;
#18778=ADVANCED_FACE ( 'NONE', ( #12848, #6771, #1709, #19290, #3485 ), #111, .T. ) ;
#18812=CARTESIAN_POINT ( 'NONE',  ( 3.600000000000060485, 10.82531754730546147, 43.00000000000000000 ) ) ;
#18856=CYLINDRICAL_SURFACE ( 'NONE', #15617, 17.50000000000000355 ) ;
#18867=CARTESIAN_POINT ( 'NONE',  ( 0.000000000000000000, 0.000000000000000000, 126.0000000000000000 ) ) ;
#18887=( NAMED_UNIT ( * ) PLANE_ANGLE_UNIT ( ) SI_UNIT ( $, .RADIAN. ) );
#18969=CARTESIAN_POINT ( 'NONE',  ( 7.500000000000000000, 9.184850993605147944E-16, 126.0000000000000000 ) ) ;
#18976=VERTEX_POINT ( 'NONE', #18969 ) ;
#18979=AXIS2_PLACEMENT_3D ( 'NONE', #4174, #15514, #6073 ) ;
#19084=DIRECTION ( 'NONE',  ( 0.000000000000000000, 0.000000000000000000, 1.000000000000000000 ) ) ;
#19171=CIRCLE ( 'NONE', #5955, 2.649999999999987477 ) ;
#19183=CARTESIAN_POINT ( 'NONE',  ( 17.50000000000000355, 2.143131898507868643E-15, 43.00000000000000000 ) ) ;
#19193=AXIS2_PLACEMENT_3D ( 'NONE', #17383, #1288, #9115 ) ;
#19195=CARTESIAN_POINT ( 'NONE',  ( 0.000000000000000000, 0.000000000000000000, 43.00000000000000000 ) ) ;
#19204=VECTOR ( 'NONE', #20939, 1000.000000000000000 ) ;
#19242=DIRECTION ( 'NONE',  ( -0.000000000000000000, -0.000000000000000000, -1.000000000000000000 ) ) ;
#19248=ORIENTED_EDGE ( 'NONE', *, *, #4734, .T. ) ;
#19263=( NAMED_UNIT ( * ) SI_UNIT ( $, .STERADIAN. ) SOLID_ANGLE_UNIT ( ) );
#19290=FACE_BOUND ( 'NONE', #3440, .T. ) ;
#19327=CARTESIAN_POINT ( 'NONE',  ( 8.900000000000046541, 10.82531754730546147, 129.0000000000000000 ) ) ;
#19330=EDGE_CURVE ( 'NONE', #7692, #16592, #19171, .T. ) ;
#19364=SHAPE_DEFINITION_REPRESENTATION ( #5258, #8160 ) ;
#19443=DIRECTION ( 'NONE',  ( -0.000000000000000000, -0.000000000000000000, 1.000000000000000000 ) ) ;
#19469=DIRECTION ( 'NONE',  ( -0.000000000000000000, -0.000000000000000000, -1.000000000000000000 ) ) ;
#19474=CARTESIAN_POINT ( 'NONE',  ( 0.000000000000000000, 0.000000000000000000, 0.000000000000000000 ) ) ;
#19532=DIRECTION ( 'NONE',  ( -0.000000000000000000, -0.000000000000000000, 1.000000000000000000 ) ) ;
#19547=CARTESIAN_POINT ( 'NONE',  ( 6.250000000000054179, 10.82531754730546147, 126.0000000000000000 ) ) ;
#19566=CARTESIAN_POINT ( 'NONE',  ( 3.600000000000060485, 10.82531754730546147, 129.0000000000000000 ) ) ;
#19578=FACE_OUTER_BOUND ( 'NONE', #14316, .T. ) ;
#19621=ORIENTED_EDGE ( 'NONE', *, *, #4964, .T. ) ;
#19623=CARTESIAN_POINT ( 'NONE',  ( 6.249999999999902300, -10.82531754730554496, 46.00000000000000711 ) ) ;
#19625=DIRECTION ( 'NONE',  ( 1.000000000000000000, 0.000000000000000000, 0.000000000000000000 ) ) ;
#19649=FACE_OUTER_BOUND ( 'NONE', #6722, .T. ) ;
#19659=ADVANCED_FACE ( 'NONE', ( #2040 ), #8296, .F. ) ;
#19697=DIRECTION ( 'NONE',  ( -0.000000000000000000, -0.000000000000000000, 1.000000000000000000 ) ) ;
#19732=CYLINDRICAL_SURFACE ( 'NONE', #18634, 2.649999999999993694 ) ;
#19738=ADVANCED_FACE ( 'NONE', ( #14313, #9524, #15784, #17595 ), #20754, .F. ) ;
#19863=VERTEX_POINT ( 'NONE', #16298 ) ;
#19870=VERTEX_POINT ( 'NONE', #14614 ) ;
#19883=CARTESIAN_POINT ( 'NONE',  ( 0.000000000000000000, 0.000000000000000000, 129.0000000000000000 ) ) ;
#19890=DIRECTION ( 'NONE',  ( 0.000000000000000000, 0.000000000000000000, 1.000000000000000000 ) ) ;
#19917=DIRECTION ( 'NONE',  ( 0.000000000000000000, 0.000000000000000000, 1.000000000000000000 ) ) ;
#19920=ORIENTED_EDGE ( 'NONE', *, *, #6864, .T. ) ;
#19947=ADVANCED_FACE ( 'NONE', ( #15338 ), #11742, .F. ) ;
#19953=CARTESIAN_POINT ( 'NONE',  ( 0.000000000000000000, 0.000000000000000000, 126.0000000000000000 ) ) ;
#19956=ORIENTED_EDGE ( 'NONE', *, *, #5871, .T. ) ;
#20054=CARTESIAN_POINT ( 'NONE',  ( 6.249999999999902300, -10.82531754730554496, 46.00000000000000711 ) ) ;
#20076=CIRCLE ( 'NONE', #5535, 2.649999999999992806 ) ;
#20108=EDGE_CURVE ( 'NONE', #2027, #16324, #1262, .T. ) ;
#20110=CARTESIAN_POINT ( 'NONE',  ( 8.899999999999895550, -10.82531754730554496, 129.0000000000000000 ) ) ;
#20141=ORIENTED_EDGE ( 'NONE', *, *, #9467, .F. ) ;
#20183=EDGE_CURVE ( 'NONE', #11488, #14272, #12425, .T. ) ;
#20197=DIRECTION ( 'NONE',  ( -0.000000000000000000, -0.000000000000000000, -1.000000000000000000 ) ) ;
#20208=ORIENTED_EDGE ( 'NONE', *, *, #8181, .T. ) ;
#20218=AXIS2_PLACEMENT_3D ( 'NONE', #18867, #4340, #10705 ) ;
#20239=EDGE_CURVE ( 'NONE', #1536, #18341, #169, .T. ) ;
#20248=FILL_AREA_STYLE ('',( #5720 ) ) ;
#20283=CARTESIAN_POINT ( 'NONE',  ( -12.50000000000000533, 0.000000000000000000, 126.0000000000000000 ) ) ;
#20338=CIRCLE ( 'NONE', #18657, 2.649999999999992806 ) ;
#20342=( LENGTH_UNIT ( ) NAMED_UNIT ( * ) SI_UNIT ( .MILLI., .METRE. ) );
#20379=CARTESIAN_POINT ( 'NONE',  ( 6.249999999999902300, -10.82531754730554496, 43.00000000000000000 ) ) ;
#20382=ADVANCED_FACE ( 'NONE', ( #17097, #13423, #10524, #5351 ), #10639, .F. ) ;
#20385=ORIENTED_EDGE ( 'NONE', *, *, #17299, .T. ) ;
#20407=CIRCLE ( 'NONE', #12288, 2.649999999999994582 ) ;
#20431=CIRCLE ( 'NONE', #2836, 2.649999999999988365 ) ;
#20662=ADVANCED_FACE ( 'NONE', ( #11966 ), #4228, .T. ) ;
#20669=CARTESIAN_POINT ( 'NONE',  ( -12.50000000000000533, 0.000000000000000000, 46.00000000000000711 ) ) ;
#20691=AXIS2_PLACEMENT_3D ( 'NONE', #13451, #18311, #16518 ) ;
#20716=DIRECTION ( 'NONE',  ( 0.000000000000000000, 0.000000000000000000, 1.000000000000000000 ) ) ;
#20754=PLANE ( 'NONE',  #19193 ) ;
#20757=ORIENTED_EDGE ( 'NONE', *, *, #5871, .F. ) ;
#20792=CARTESIAN_POINT ( 'NONE',  ( 3.600000000000060485, 10.82531754730546147, 126.0000000000000000 ) ) ;
#20827=AXIS2_PLACEMENT_3D ( 'NONE', #8826, #1427, #4703 ) ;
#20839=VERTEX_POINT ( 'NONE', #6433 ) ;
#20869=CARTESIAN_POINT ( 'NONE',  ( 7.500000000000000000, 9.184850993605147944E-16, 46.00000000000000711 ) ) ;
#20889=ADVANCED_FACE ( 'NONE', ( #19578 ), #13332, .T. ) ;
#20892=FACE_OUTER_BOUND ( 'NONE', #16520, .T. ) ;
#20938=ORIENTED_EDGE ( 'NONE', *, *, #3374, .F. ) ;
#20939=DIRECTION ( 'NONE',  ( -0.000000000000000000, -0.000000000000000000, 1.000000000000000000 ) ) ;
ENDSEC;
END-ISO-10303-21;
